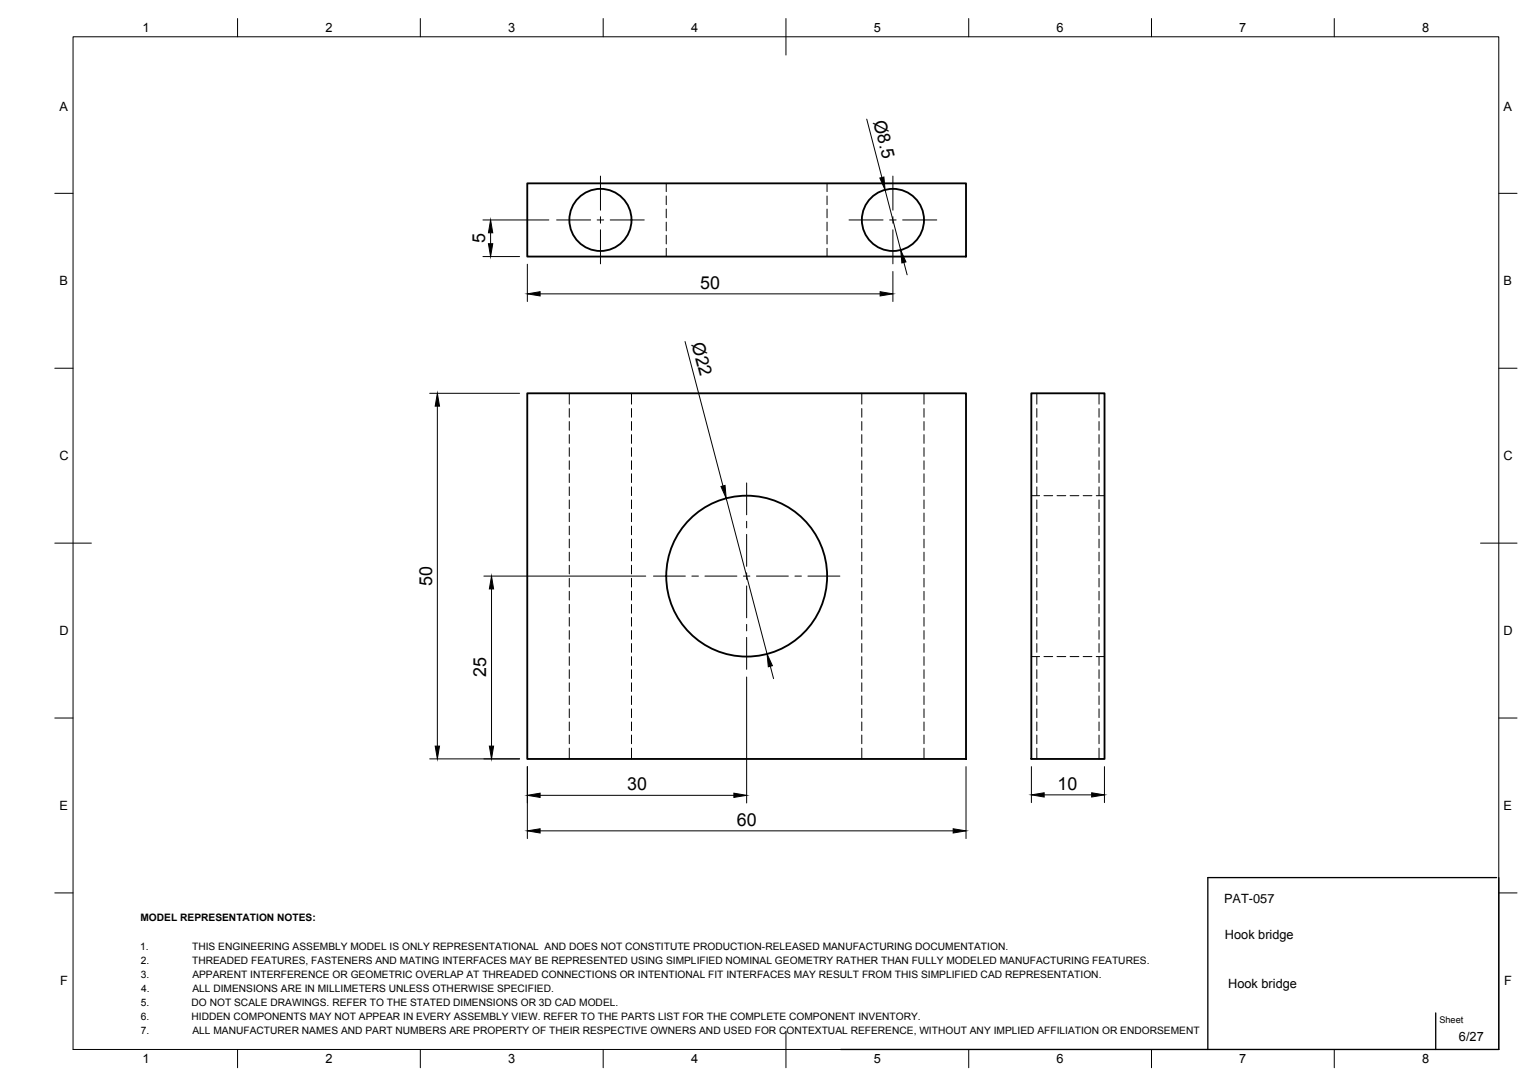
ISO-10303-21;
HEADER;
/* Generated by software containing ST-Developer
 * from STEP Tools, Inc. (www.steptools.com) 
 */

FILE_DESCRIPTION(
/* description */ ('Bearing-mounted hook block'),
/* implementation_level */ '2;1');

FILE_NAME(
/* name */ 'Hook bridge.step',
/* time_stamp */ '2026-10-28T22:30:11-07:00',
/* author */ (''),
/* organization */ (''),
/* preprocessor_version */ 'ST-DEVELOPER v20.2',
/* originating_system */ 'Autodesk Translation Framework v15.17.0.0',
/* authorisation */ '');

FILE_SCHEMA (('AUTOMOTIVE_DESIGN { 1 0 10303 214 3 1 1 }'));
ENDSEC;

DATA;
#10=MECHANICAL_DESIGN_GEOMETRIC_PRESENTATION_REPRESENTATION('',(#324),#7609);
#276=SHAPE_REPRESENTATION_RELATIONSHIP('SRR','None',#7723,#300);
#300=ADVANCED_BREP_SHAPE_REPRESENTATION('',(#356),#7583);
#324=STYLED_ITEM('',(#7945),#356);
#356=MANIFOLD_SOLID_BREP('Body1',#3920);
#425=LINE('',#6221,#655);
#426=LINE('',#6227,#656);
#427=LINE('',#6233,#657);
#428=LINE('',#6238,#658);
#429=LINE('',#6240,#659);
#430=LINE('',#6242,#660);
#431=LINE('',#6243,#661);
#432=LINE('',#6246,#662);
#433=LINE('',#6248,#663);
#434=LINE('',#6249,#664);
#435=LINE('',#6252,#665);
#436=LINE('',#6254,#666);
#437=LINE('',#6255,#667);
#438=LINE('',#6257,#668);
#439=LINE('',#6258,#669);
#655=VECTOR('',#4928,1.1);
#656=VECTOR('',#4935,0.425);
#657=VECTOR('',#4942,0.425);
#658=VECTOR('',#4947,1.);
#659=VECTOR('',#4948,1.);
#660=VECTOR('',#4949,1.);
#661=VECTOR('',#4950,1.);
#662=VECTOR('',#4953,1.);
#663=VECTOR('',#4954,1.);
#664=VECTOR('',#4955,1.);
#665=VECTOR('',#4958,1.);
#666=VECTOR('',#4959,1.);
#667=VECTOR('',#4960,1.);
#668=VECTOR('',#4963,1.);
#669=VECTOR('',#4964,1.);
#857=CYLINDRICAL_SURFACE('',#4282,1.1);
#858=CYLINDRICAL_SURFACE('',#4285,0.425);
#859=CYLINDRICAL_SURFACE('',#4288,0.425);
#935=FACE_BOUND('',#1280,.T.);
#936=FACE_BOUND('',#1281,.T.);
#937=FACE_BOUND('',#1284,.T.);
#938=FACE_BOUND('',#1285,.T.);
#939=FACE_BOUND('',#1288,.T.);
#940=FACE_BOUND('',#1290,.T.);
#1026=FACE_OUTER_BOUND('',#1276,.T.);
#1027=FACE_OUTER_BOUND('',#1277,.T.);
#1028=FACE_OUTER_BOUND('',#1278,.T.);
#1029=FACE_OUTER_BOUND('',#1279,.T.);
#1030=FACE_OUTER_BOUND('',#1282,.T.);
#1031=FACE_OUTER_BOUND('',#1283,.T.);
#1032=FACE_OUTER_BOUND('',#1286,.T.);
#1033=FACE_OUTER_BOUND('',#1287,.T.);
#1034=FACE_OUTER_BOUND('',#1289,.T.);
#1276=EDGE_LOOP('',(#2740,#2741,#2742,#2743));
#1277=EDGE_LOOP('',(#2744,#2745,#2746,#2747));
#1278=EDGE_LOOP('',(#2748,#2749,#2750,#2751));
#1279=EDGE_LOOP('',(#2752,#2753,#2754,#2755));
#1280=EDGE_LOOP('',(#2756));
#1281=EDGE_LOOP('',(#2757));
#1282=EDGE_LOOP('',(#2758,#2759,#2760,#2761));
#1283=EDGE_LOOP('',(#2762,#2763,#2764,#2765));
#1284=EDGE_LOOP('',(#2766));
#1285=EDGE_LOOP('',(#2767));
#1286=EDGE_LOOP('',(#2768,#2769,#2770,#2771));
#1287=EDGE_LOOP('',(#2772,#2773,#2774,#2775));
#1288=EDGE_LOOP('',(#2776));
#1289=EDGE_LOOP('',(#2777,#2778,#2779,#2780));
#1290=EDGE_LOOP('',(#2781));
#1587=CIRCLE('',#4283,1.1);
#1588=CIRCLE('',#4284,1.1);
#1589=CIRCLE('',#4286,0.425);
#1590=CIRCLE('',#4287,0.425);
#1591=CIRCLE('',#4289,0.425);
#1592=CIRCLE('',#4290,0.425);
#1828=VERTEX_POINT('',#6218);
#1829=VERTEX_POINT('',#6220);
#1830=VERTEX_POINT('',#6224);
#1831=VERTEX_POINT('',#6226);
#1832=VERTEX_POINT('',#6230);
#1833=VERTEX_POINT('',#6232);
#1834=VERTEX_POINT('',#6236);
#1835=VERTEX_POINT('',#6237);
#1836=VERTEX_POINT('',#6239);
#1837=VERTEX_POINT('',#6241);
#1838=VERTEX_POINT('',#6245);
#1839=VERTEX_POINT('',#6247);
#1840=VERTEX_POINT('',#6251);
#1841=VERTEX_POINT('',#6253);
#2180=EDGE_CURVE('',#1828,#1828,#1587,.T.);
#2181=EDGE_CURVE('',#1828,#1829,#425,.T.);
#2182=EDGE_CURVE('',#1829,#1829,#1588,.T.);
#2183=EDGE_CURVE('',#1830,#1830,#1589,.T.);
#2184=EDGE_CURVE('',#1830,#1831,#426,.T.);
#2185=EDGE_CURVE('',#1831,#1831,#1590,.T.);
#2186=EDGE_CURVE('',#1832,#1832,#1591,.T.);
#2187=EDGE_CURVE('',#1832,#1833,#427,.T.);
#2188=EDGE_CURVE('',#1833,#1833,#1592,.T.);
#2189=EDGE_CURVE('',#1834,#1835,#428,.T.);
#2190=EDGE_CURVE('',#1835,#1836,#429,.T.);
#2191=EDGE_CURVE('',#1837,#1836,#430,.T.);
#2192=EDGE_CURVE('',#1834,#1837,#431,.T.);
#2193=EDGE_CURVE('',#1838,#1834,#432,.T.);
#2194=EDGE_CURVE('',#1839,#1837,#433,.T.);
#2195=EDGE_CURVE('',#1838,#1839,#434,.T.);
#2196=EDGE_CURVE('',#1840,#1838,#435,.T.);
#2197=EDGE_CURVE('',#1841,#1839,#436,.T.);
#2198=EDGE_CURVE('',#1840,#1841,#437,.T.);
#2199=EDGE_CURVE('',#1835,#1840,#438,.T.);
#2200=EDGE_CURVE('',#1836,#1841,#439,.T.);
#2740=ORIENTED_EDGE('',*,*,#2180,.F.);
#2741=ORIENTED_EDGE('',*,*,#2181,.T.);
#2742=ORIENTED_EDGE('',*,*,#2182,.F.);
#2743=ORIENTED_EDGE('',*,*,#2181,.F.);
#2744=ORIENTED_EDGE('',*,*,#2183,.F.);
#2745=ORIENTED_EDGE('',*,*,#2184,.T.);
#2746=ORIENTED_EDGE('',*,*,#2185,.F.);
#2747=ORIENTED_EDGE('',*,*,#2184,.F.);
#2748=ORIENTED_EDGE('',*,*,#2186,.F.);
#2749=ORIENTED_EDGE('',*,*,#2187,.T.);
#2750=ORIENTED_EDGE('',*,*,#2188,.F.);
#2751=ORIENTED_EDGE('',*,*,#2187,.F.);
#2752=ORIENTED_EDGE('',*,*,#2189,.T.);
#2753=ORIENTED_EDGE('',*,*,#2190,.T.);
#2754=ORIENTED_EDGE('',*,*,#2191,.F.);
#2755=ORIENTED_EDGE('',*,*,#2192,.F.);
#2756=ORIENTED_EDGE('',*,*,#2185,.T.);
#2757=ORIENTED_EDGE('',*,*,#2188,.T.);
#2758=ORIENTED_EDGE('',*,*,#2193,.T.);
#2759=ORIENTED_EDGE('',*,*,#2192,.T.);
#2760=ORIENTED_EDGE('',*,*,#2194,.F.);
#2761=ORIENTED_EDGE('',*,*,#2195,.F.);
#2762=ORIENTED_EDGE('',*,*,#2196,.T.);
#2763=ORIENTED_EDGE('',*,*,#2195,.T.);
#2764=ORIENTED_EDGE('',*,*,#2197,.F.);
#2765=ORIENTED_EDGE('',*,*,#2198,.F.);
#2766=ORIENTED_EDGE('',*,*,#2183,.T.);
#2767=ORIENTED_EDGE('',*,*,#2186,.T.);
#2768=ORIENTED_EDGE('',*,*,#2199,.T.);
#2769=ORIENTED_EDGE('',*,*,#2198,.T.);
#2770=ORIENTED_EDGE('',*,*,#2200,.F.);
#2771=ORIENTED_EDGE('',*,*,#2190,.F.);
#2772=ORIENTED_EDGE('',*,*,#2200,.T.);
#2773=ORIENTED_EDGE('',*,*,#2197,.T.);
#2774=ORIENTED_EDGE('',*,*,#2194,.T.);
#2775=ORIENTED_EDGE('',*,*,#2191,.T.);
#2776=ORIENTED_EDGE('',*,*,#2182,.T.);
#2777=ORIENTED_EDGE('',*,*,#2199,.F.);
#2778=ORIENTED_EDGE('',*,*,#2189,.F.);
#2779=ORIENTED_EDGE('',*,*,#2193,.F.);
#2780=ORIENTED_EDGE('',*,*,#2196,.F.);
#2781=ORIENTED_EDGE('',*,*,#2180,.T.);
#3572=PLANE('',#4291);
#3573=PLANE('',#4292);
#3574=PLANE('',#4293);
#3575=PLANE('',#4294);
#3576=PLANE('',#4295);
#3577=PLANE('',#4296);
#3708=ADVANCED_FACE('',(#1026),#857,.F.);
#3709=ADVANCED_FACE('',(#1027),#858,.F.);
#3710=ADVANCED_FACE('',(#1028),#859,.F.);
#3711=ADVANCED_FACE('',(#1029,#935,#936),#3572,.T.);
#3712=ADVANCED_FACE('',(#1030),#3573,.T.);
#3713=ADVANCED_FACE('',(#1031,#937,#938),#3574,.T.);
#3714=ADVANCED_FACE('',(#1032),#3575,.T.);
#3715=ADVANCED_FACE('',(#1033,#939),#3576,.T.);
#3716=ADVANCED_FACE('',(#1034,#940),#3577,.F.);
#3920=CLOSED_SHELL('',(#3708,#3709,#3710,#3711,#3712,#3713,#3714,#3715,
#3716));
#4281=AXIS2_PLACEMENT_3D('',#6216,#4922,#4923);
#4282=AXIS2_PLACEMENT_3D('',#6217,#4924,#4925);
#4283=AXIS2_PLACEMENT_3D('',#6219,#4926,#4927);
#4284=AXIS2_PLACEMENT_3D('',#6222,#4929,#4930);
#4285=AXIS2_PLACEMENT_3D('',#6223,#4931,#4932);
#4286=AXIS2_PLACEMENT_3D('',#6225,#4933,#4934);
#4287=AXIS2_PLACEMENT_3D('',#6228,#4936,#4937);
#4288=AXIS2_PLACEMENT_3D('',#6229,#4938,#4939);
#4289=AXIS2_PLACEMENT_3D('',#6231,#4940,#4941);
#4290=AXIS2_PLACEMENT_3D('',#6234,#4943,#4944);
#4291=AXIS2_PLACEMENT_3D('',#6235,#4945,#4946);
#4292=AXIS2_PLACEMENT_3D('',#6244,#4951,#4952);
#4293=AXIS2_PLACEMENT_3D('',#6250,#4956,#4957);
#4294=AXIS2_PLACEMENT_3D('',#6256,#4961,#4962);
#4295=AXIS2_PLACEMENT_3D('',#6259,#4965,#4966);
#4296=AXIS2_PLACEMENT_3D('',#6260,#4967,#4968);
#4922=DIRECTION('axis',(0.,0.,1.));
#4923=DIRECTION('refdir',(1.,0.,0.));
#4924=DIRECTION('center_axis',(0.,0.,1.));
#4925=DIRECTION('ref_axis',(1.,0.,0.));
#4926=DIRECTION('center_axis',(0.,0.,1.));
#4927=DIRECTION('ref_axis',(1.,0.,0.));
#4928=DIRECTION('',(0.,0.,1.));
#4929=DIRECTION('center_axis',(0.,0.,-1.));
#4930=DIRECTION('ref_axis',(1.,0.,0.));
#4931=DIRECTION('center_axis',(0.,1.,0.));
#4932=DIRECTION('ref_axis',(1.,0.,0.));
#4933=DIRECTION('center_axis',(0.,1.,0.));
#4934=DIRECTION('ref_axis',(1.,0.,0.));
#4935=DIRECTION('',(0.,1.,0.));
#4936=DIRECTION('center_axis',(0.,-1.,0.));
#4937=DIRECTION('ref_axis',(1.,0.,0.));
#4938=DIRECTION('center_axis',(0.,1.,0.));
#4939=DIRECTION('ref_axis',(1.,0.,0.));
#4940=DIRECTION('center_axis',(0.,1.,0.));
#4941=DIRECTION('ref_axis',(1.,0.,0.));
#4942=DIRECTION('',(0.,1.,0.));
#4943=DIRECTION('center_axis',(0.,-1.,0.));
#4944=DIRECTION('ref_axis',(1.,0.,0.));
#4945=DIRECTION('center_axis',(0.,1.,0.));
#4946=DIRECTION('ref_axis',(-1.,0.,0.));
#4947=DIRECTION('',(-1.,0.,0.));
#4948=DIRECTION('',(0.,0.,1.));
#4949=DIRECTION('',(-1.,0.,0.));
#4950=DIRECTION('',(0.,0.,1.));
#4951=DIRECTION('center_axis',(1.,0.,0.));
#4952=DIRECTION('ref_axis',(0.,1.,0.));
#4953=DIRECTION('',(0.,1.,0.));
#4954=DIRECTION('',(0.,1.,0.));
#4955=DIRECTION('',(0.,0.,1.));
#4956=DIRECTION('center_axis',(0.,-1.,0.));
#4957=DIRECTION('ref_axis',(1.,0.,0.));
#4958=DIRECTION('',(1.,0.,0.));
#4959=DIRECTION('',(1.,0.,0.));
#4960=DIRECTION('',(0.,0.,1.));
#4961=DIRECTION('center_axis',(-1.,0.,0.));
#4962=DIRECTION('ref_axis',(0.,-1.,0.));
#4963=DIRECTION('',(0.,-1.,0.));
#4964=DIRECTION('',(0.,-1.,0.));
#4965=DIRECTION('center_axis',(0.,0.,1.));
#4966=DIRECTION('ref_axis',(1.,0.,0.));
#4967=DIRECTION('center_axis',(0.,0.,1.));
#4968=DIRECTION('ref_axis',(1.,0.,0.));
#6216=CARTESIAN_POINT('',(0.,0.,0.));
#6217=CARTESIAN_POINT('Origin',(0.,0.,4.4));
#6218=CARTESIAN_POINT('',(-1.1,-1.34711147906209E-16,4.5));
#6219=CARTESIAN_POINT('Origin',(0.,0.,4.5));
#6220=CARTESIAN_POINT('',(-1.1,1.34711147906209E-16,5.5));
#6221=CARTESIAN_POINT('',(-1.1,-1.34711147906209E-16,4.4));
#6222=CARTESIAN_POINT('Origin',(0.,0.,5.5));
#6223=CARTESIAN_POINT('Origin',(-2.,-2.6,5.));
#6224=CARTESIAN_POINT('',(-2.425,-2.5,5.));
#6225=CARTESIAN_POINT('Origin',(-2.,-2.5,5.));
#6226=CARTESIAN_POINT('',(-2.425,2.5,5.));
#6227=CARTESIAN_POINT('',(-2.425,-2.6,5.));
#6228=CARTESIAN_POINT('Origin',(-2.,2.5,5.));
#6229=CARTESIAN_POINT('Origin',(2.,-2.6,5.));
#6230=CARTESIAN_POINT('',(1.575,-2.5,5.));
#6231=CARTESIAN_POINT('Origin',(2.,-2.5,5.));
#6232=CARTESIAN_POINT('',(1.575,2.5,5.));
#6233=CARTESIAN_POINT('',(1.575,-2.6,5.));
#6234=CARTESIAN_POINT('Origin',(2.,2.5,5.));
#6235=CARTESIAN_POINT('Origin',(3.,2.5,4.5));
#6236=CARTESIAN_POINT('',(3.,2.5,4.5));
#6237=CARTESIAN_POINT('',(-3.,2.5,4.5));
#6238=CARTESIAN_POINT('',(3.,2.5,4.5));
#6239=CARTESIAN_POINT('',(-3.,2.5,5.5));
#6240=CARTESIAN_POINT('',(-3.,2.5,4.5));
#6241=CARTESIAN_POINT('',(3.,2.5,5.5));
#6242=CARTESIAN_POINT('',(3.,2.5,5.5));
#6243=CARTESIAN_POINT('',(3.,2.5,4.5));
#6244=CARTESIAN_POINT('Origin',(3.,-2.5,4.5));
#6245=CARTESIAN_POINT('',(3.,-2.5,4.5));
#6246=CARTESIAN_POINT('',(3.,-2.5,4.5));
#6247=CARTESIAN_POINT('',(3.,-2.5,5.5));
#6248=CARTESIAN_POINT('',(3.,-2.5,5.5));
#6249=CARTESIAN_POINT('',(3.,-2.5,4.5));
#6250=CARTESIAN_POINT('Origin',(-3.,-2.5,4.5));
#6251=CARTESIAN_POINT('',(-3.,-2.5,4.5));
#6252=CARTESIAN_POINT('',(-3.,-2.5,4.5));
#6253=CARTESIAN_POINT('',(-3.,-2.5,5.5));
#6254=CARTESIAN_POINT('',(-3.,-2.5,5.5));
#6255=CARTESIAN_POINT('',(-3.,-2.5,4.5));
#6256=CARTESIAN_POINT('Origin',(-3.,2.5,4.5));
#6257=CARTESIAN_POINT('',(-3.,2.5,4.5));
#6258=CARTESIAN_POINT('',(-3.,2.5,5.5));
#6259=CARTESIAN_POINT('Origin',(0.,0.,5.5));
#6260=CARTESIAN_POINT('Origin',(0.,0.,4.5));
#7553=UNCERTAINTY_MEASURE_WITH_UNIT(LENGTH_MEASURE(0.001),#7610,
'DISTANCE_ACCURACY_VALUE',
'Maximum model space distance between geometric entities at asserted c
onnectivities');
#7579=UNCERTAINTY_MEASURE_WITH_UNIT(LENGTH_MEASURE(0.001),#7610,
'DISTANCE_ACCURACY_VALUE',
'Maximum model space distance between geometric entities at asserted c
onnectivities');
#7583=(
GEOMETRIC_REPRESENTATION_CONTEXT(3)
GLOBAL_UNCERTAINTY_ASSIGNED_CONTEXT((#7553))
GLOBAL_UNIT_ASSIGNED_CONTEXT((#7610,#7612,#7613))
REPRESENTATION_CONTEXT('','3D')
);
#7609=(
GEOMETRIC_REPRESENTATION_CONTEXT(3)
GLOBAL_UNCERTAINTY_ASSIGNED_CONTEXT((#7579))
GLOBAL_UNIT_ASSIGNED_CONTEXT((#7610,#7612,#7613))
REPRESENTATION_CONTEXT('','3D')
);
#7610=(
LENGTH_UNIT()
NAMED_UNIT(*)
SI_UNIT(.CENTI.,.METRE.)
);
#7612=(
NAMED_UNIT(*)
PLANE_ANGLE_UNIT()
SI_UNIT($,.RADIAN.)
);
#7613=(
NAMED_UNIT(*)
SI_UNIT($,.STERADIAN.)
SOLID_ANGLE_UNIT()
);
#7617=SHAPE_DEFINITION_REPRESENTATION(#7646,#7723);
#7646=PRODUCT_DEFINITION_SHAPE('',$,#7753);
#7723=SHAPE_REPRESENTATION('',(#4281),#7583);
#7749=PRODUCT_DEFINITION_CONTEXT('part definition',#7838,'design');
#7753=PRODUCT_DEFINITION('Hook bridge','Hook bridge',#7782,#7749);
#7782=PRODUCT_DEFINITION_FORMATION('',$,#7843);
#7838=APPLICATION_CONTEXT(
'Core Data for Automotive Mechanical Design Process');
#7839=PRODUCT_CONTEXT('part definition',#7838,'mechanical');
#7843=PRODUCT('Hook bridge','Hook bridge','Hook bridge',(#7839));
#7939=COLOUR_RGB('Off White',0.89,0.88,0.83);
#7940=FILL_AREA_STYLE_COLOUR('',#7939);
#7941=FILL_AREA_STYLE('',(#7940));
#7942=SURFACE_STYLE_FILL_AREA(#7941);
#7943=SURFACE_SIDE_STYLE('',(#7942));
#7944=SURFACE_STYLE_USAGE(.BOTH.,#7943);
#7945=PRESENTATION_STYLE_ASSIGNMENT((#7944));
ENDSEC;
END-ISO-10303-21;
